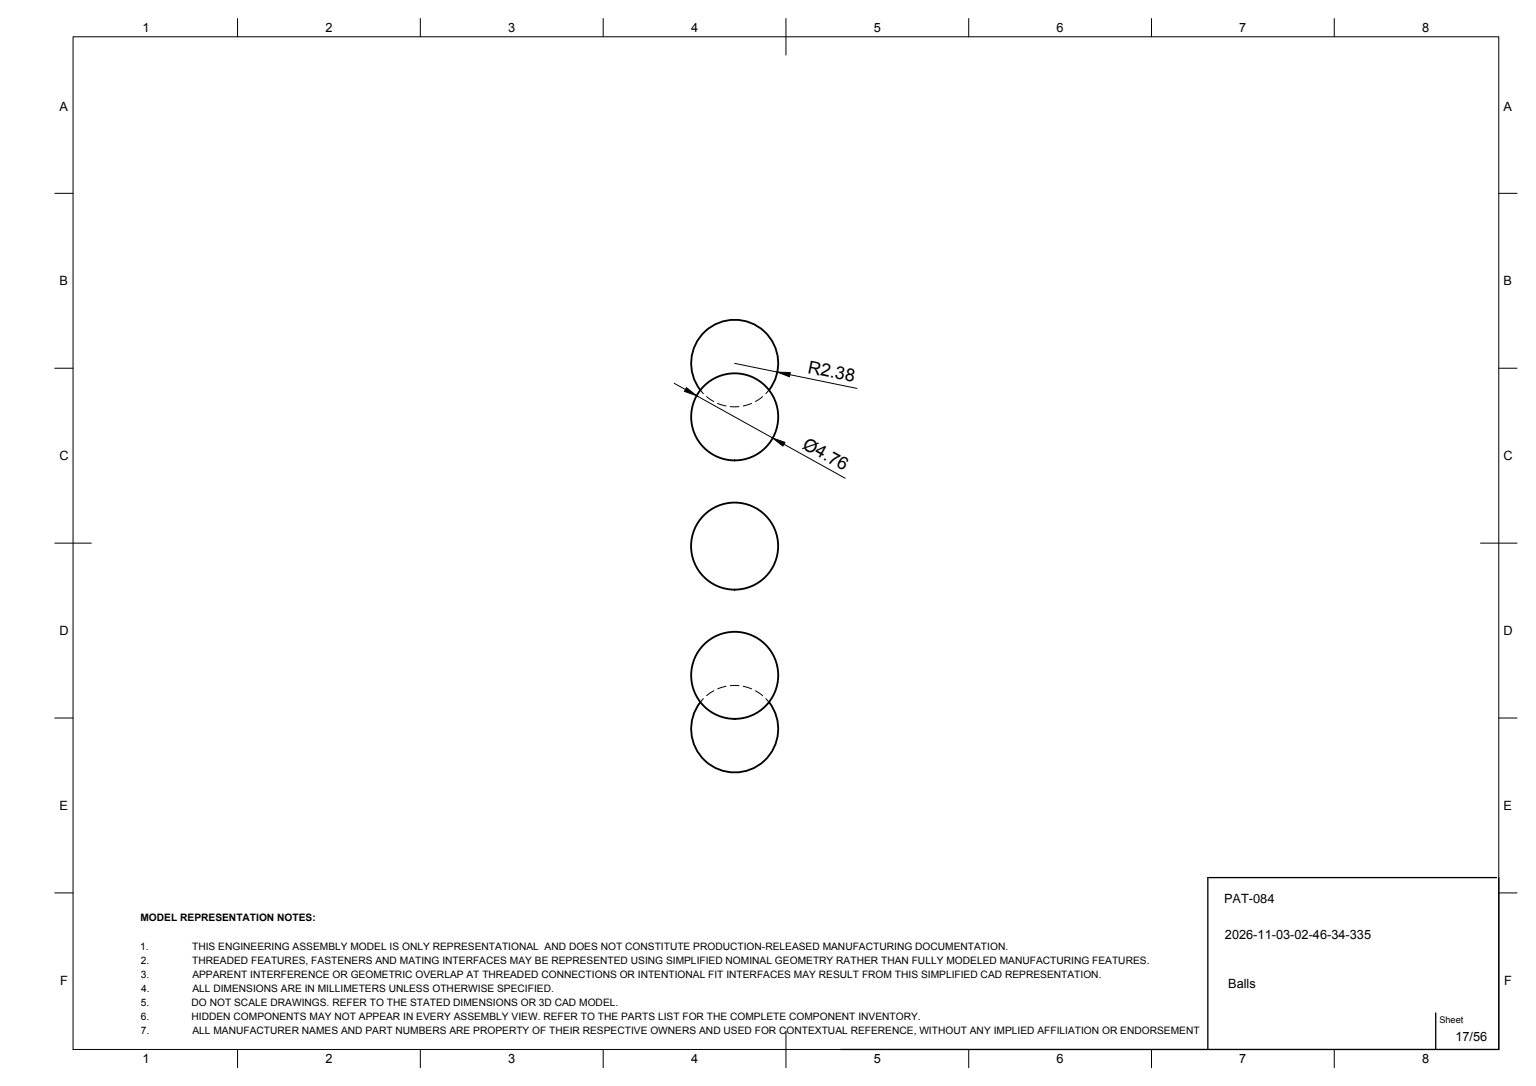
ISO-10303-21;
HEADER;
/* Generated by software containing ST-Developer
 * from STEP Tools, Inc. (www.steptools.com) 
 */

FILE_DESCRIPTION(
/* description */ ('Quick-return (Whitworth) mechanism'),
/* implementation_level */ '2;1');

FILE_NAME(
/* name */ 'Balls.step',
/* time_stamp */ '2026-10-28T03:25:57-07:00',
/* author */ (''),
/* organization */ (''),
/* preprocessor_version */ 'ST-DEVELOPER v20.2',
/* originating_system */ 'Autodesk Translation Framework v15.17.0.0',
/* authorisation */ '');

FILE_SCHEMA (('AUTOMOTIVE_DESIGN { 1 0 10303 214 3 1 1 }'));
ENDSEC;

DATA;
#10=MECHANICAL_DESIGN_GEOMETRIC_PRESENTATION_REPRESENTATION('',(#500,#501,#502,#503,#504,#505,#506,#507),#14878);
#333=SPHERICAL_SURFACE('',#8750,0.23815);
#334=SPHERICAL_SURFACE('',#8752,0.23815);
#335=SPHERICAL_SURFACE('',#8754,0.23815);
#336=SPHERICAL_SURFACE('',#8756,0.23815);
#337=SPHERICAL_SURFACE('',#8758,0.23815);
#338=SPHERICAL_SURFACE('',#8760,0.23815);
#339=SPHERICAL_SURFACE('',#8762,0.23815);
#340=SPHERICAL_SURFACE('',#8764,0.23815);
#412=SHAPE_REPRESENTATION_RELATIONSHIP('SRR','None',#15081,#456);
#456=ADVANCED_BREP_SHAPE_REPRESENTATION('',(#552,#553,#554,#555,#556,#557,
#558,#559),#14838);
#500=STYLED_ITEM('',(#15406),#552);
#501=STYLED_ITEM('',(#15406),#553);
#502=STYLED_ITEM('',(#15406),#554);
#503=STYLED_ITEM('',(#15406),#555);
#504=STYLED_ITEM('',(#15406),#556);
#505=STYLED_ITEM('',(#15406),#557);
#506=STYLED_ITEM('',(#15406),#558);
#507=STYLED_ITEM('',(#15406),#559);
#552=MANIFOLD_SOLID_BREP('Body1',#7854);
#553=MANIFOLD_SOLID_BREP('Body2',#7855);
#554=MANIFOLD_SOLID_BREP('Body3',#7856);
#555=MANIFOLD_SOLID_BREP('Body4',#7857);
#556=MANIFOLD_SOLID_BREP('Body5',#7858);
#557=MANIFOLD_SOLID_BREP('Body6',#7859);
#558=MANIFOLD_SOLID_BREP('Body7',#7860);
#559=MANIFOLD_SOLID_BREP('Body8',#7861);
#1213=FACE_OUTER_BOUND('',#1785,.T.);
#1214=FACE_OUTER_BOUND('',#1786,.T.);
#1215=FACE_OUTER_BOUND('',#1787,.T.);
#1216=FACE_OUTER_BOUND('',#1788,.T.);
#1217=FACE_OUTER_BOUND('',#1789,.T.);
#1218=FACE_OUTER_BOUND('',#1790,.T.);
#1219=FACE_OUTER_BOUND('',#1791,.T.);
#1220=FACE_OUTER_BOUND('',#1792,.T.);
#1785=EDGE_LOOP('',(#5982,#5983));
#1786=EDGE_LOOP('',(#5984,#5985));
#1787=EDGE_LOOP('',(#5986,#5987));
#1788=EDGE_LOOP('',(#5988,#5989));
#1789=EDGE_LOOP('',(#5990,#5991));
#1790=EDGE_LOOP('',(#5992,#5993));
#1791=EDGE_LOOP('',(#5994,#5995));
#1792=EDGE_LOOP('',(#5996,#5997));
#3402=CIRCLE('',#8751,0.23815);
#3403=CIRCLE('',#8753,0.23815);
#3404=CIRCLE('',#8755,0.23815);
#3405=CIRCLE('',#8757,0.23815);
#3406=CIRCLE('',#8759,0.23815);
#3407=CIRCLE('',#8761,0.23815);
#3408=CIRCLE('',#8763,0.23815);
#3409=CIRCLE('',#8765,0.23815);
#3871=VERTEX_POINT('',#12863);
#3872=VERTEX_POINT('',#12864);
#3873=VERTEX_POINT('',#12867);
#3874=VERTEX_POINT('',#12868);
#3875=VERTEX_POINT('',#12871);
#3876=VERTEX_POINT('',#12872);
#3877=VERTEX_POINT('',#12875);
#3878=VERTEX_POINT('',#12876);
#3879=VERTEX_POINT('',#12879);
#3880=VERTEX_POINT('',#12880);
#3881=VERTEX_POINT('',#12883);
#3882=VERTEX_POINT('',#12884);
#3883=VERTEX_POINT('',#12887);
#3884=VERTEX_POINT('',#12888);
#3885=VERTEX_POINT('',#12891);
#3886=VERTEX_POINT('',#12892);
#4648=EDGE_CURVE('',#3871,#3872,#3402,.T.);
#4649=EDGE_CURVE('',#3873,#3874,#3403,.T.);
#4650=EDGE_CURVE('',#3875,#3876,#3404,.T.);
#4651=EDGE_CURVE('',#3877,#3878,#3405,.T.);
#4652=EDGE_CURVE('',#3879,#3880,#3406,.T.);
#4653=EDGE_CURVE('',#3881,#3882,#3407,.T.);
#4654=EDGE_CURVE('',#3883,#3884,#3408,.T.);
#4655=EDGE_CURVE('',#3885,#3886,#3409,.T.);
#5982=ORIENTED_EDGE('',*,*,#4648,.T.);
#5983=ORIENTED_EDGE('',*,*,#4648,.F.);
#5984=ORIENTED_EDGE('',*,*,#4649,.T.);
#5985=ORIENTED_EDGE('',*,*,#4649,.F.);
#5986=ORIENTED_EDGE('',*,*,#4650,.T.);
#5987=ORIENTED_EDGE('',*,*,#4650,.F.);
#5988=ORIENTED_EDGE('',*,*,#4651,.T.);
#5989=ORIENTED_EDGE('',*,*,#4651,.F.);
#5990=ORIENTED_EDGE('',*,*,#4652,.T.);
#5991=ORIENTED_EDGE('',*,*,#4652,.F.);
#5992=ORIENTED_EDGE('',*,*,#4653,.T.);
#5993=ORIENTED_EDGE('',*,*,#4653,.F.);
#5994=ORIENTED_EDGE('',*,*,#4654,.T.);
#5995=ORIENTED_EDGE('',*,*,#4654,.F.);
#5996=ORIENTED_EDGE('',*,*,#4655,.T.);
#5997=ORIENTED_EDGE('',*,*,#4655,.F.);
#7544=ADVANCED_FACE('',(#1213),#333,.T.);
#7545=ADVANCED_FACE('',(#1214),#334,.T.);
#7546=ADVANCED_FACE('',(#1215),#335,.T.);
#7547=ADVANCED_FACE('',(#1216),#336,.T.);
#7548=ADVANCED_FACE('',(#1217),#337,.T.);
#7549=ADVANCED_FACE('',(#1218),#338,.T.);
#7550=ADVANCED_FACE('',(#1219),#339,.T.);
#7551=ADVANCED_FACE('',(#1220),#340,.T.);
#7854=CLOSED_SHELL('',(#7544));
#7855=CLOSED_SHELL('',(#7545));
#7856=CLOSED_SHELL('',(#7546));
#7857=CLOSED_SHELL('',(#7547));
#7858=CLOSED_SHELL('',(#7548));
#7859=CLOSED_SHELL('',(#7549));
#7860=CLOSED_SHELL('',(#7550));
#7861=CLOSED_SHELL('',(#7551));
#8749=AXIS2_PLACEMENT_3D('',#12861,#10293,#10294);
#8750=AXIS2_PLACEMENT_3D('',#12862,#10295,#10296);
#8751=AXIS2_PLACEMENT_3D('',#12865,#10297,#10298);
#8752=AXIS2_PLACEMENT_3D('',#12866,#10299,#10300);
#8753=AXIS2_PLACEMENT_3D('',#12869,#10301,#10302);
#8754=AXIS2_PLACEMENT_3D('',#12870,#10303,#10304);
#8755=AXIS2_PLACEMENT_3D('',#12873,#10305,#10306);
#8756=AXIS2_PLACEMENT_3D('',#12874,#10307,#10308);
#8757=AXIS2_PLACEMENT_3D('',#12877,#10309,#10310);
#8758=AXIS2_PLACEMENT_3D('',#12878,#10311,#10312);
#8759=AXIS2_PLACEMENT_3D('',#12881,#10313,#10314);
#8760=AXIS2_PLACEMENT_3D('',#12882,#10315,#10316);
#8761=AXIS2_PLACEMENT_3D('',#12885,#10317,#10318);
#8762=AXIS2_PLACEMENT_3D('',#12886,#10319,#10320);
#8763=AXIS2_PLACEMENT_3D('',#12889,#10321,#10322);
#8764=AXIS2_PLACEMENT_3D('',#12890,#10323,#10324);
#8765=AXIS2_PLACEMENT_3D('',#12893,#10325,#10326);
#10293=DIRECTION('axis',(0.,0.,1.));
#10294=DIRECTION('refdir',(1.,0.,0.));
#10295=DIRECTION('center_axis',(0.,0.,1.));
#10296=DIRECTION('ref_axis',(1.,0.,0.));
#10297=DIRECTION('center_axis',(1.22464679914735E-16,-1.,0.));
#10298=DIRECTION('ref_axis',(-1.,-1.22464679914735E-16,0.));
#10299=DIRECTION('center_axis',(0.707106781186548,0.,0.707106781186548));
#10300=DIRECTION('ref_axis',(0.707106781186548,0.,-0.707106781186548));
#10301=DIRECTION('center_axis',(8.65956056235494E-17,-1.,-8.65956056235493E-17));
#10302=DIRECTION('ref_axis',(-0.707106781186547,-1.22464679914735E-16,0.707106781186547));
#10303=DIRECTION('center_axis',(1.,0.,0.));
#10304=DIRECTION('ref_axis',(6.12323399573676E-17,0.,-1.));
#10305=DIRECTION('center_axis',(7.49879891330929E-33,-1.,-1.22464679914735E-16));
#10306=DIRECTION('ref_axis',(-6.12323399573676E-17,-1.22464679914735E-16,
1.));
#10307=DIRECTION('center_axis',(0.707106781186548,0.,-0.707106781186548));
#10308=DIRECTION('ref_axis',(-0.707106781186548,0.,-0.707106781186548));
#10309=DIRECTION('center_axis',(-8.65956056235493E-17,-1.,-8.65956056235494E-17));
#10310=DIRECTION('ref_axis',(0.707106781186547,-1.22464679914735E-16,0.707106781186547));
#10311=DIRECTION('center_axis',(0.,0.,-1.));
#10312=DIRECTION('ref_axis',(-1.,0.,-1.22464679914735E-16));
#10313=DIRECTION('center_axis',(-1.22464679914735E-16,-1.,-1.49975978266186E-32));
#10314=DIRECTION('ref_axis',(1.,-1.22464679914735E-16,1.22464679914735E-16));
#10315=DIRECTION('center_axis',(-0.707106781186547,0.,-0.707106781186548));
#10316=DIRECTION('ref_axis',(-0.707106781186548,0.,0.707106781186547));
#10317=DIRECTION('center_axis',(-8.65956056235493E-17,-1.,8.65956056235493E-17));
#10318=DIRECTION('ref_axis',(0.707106781186548,-1.22464679914735E-16,-0.707106781186547));
#10319=DIRECTION('center_axis',(-1.,0.,0.));
#10320=DIRECTION('ref_axis',(-1.83697019872103E-16,0.,1.));
#10321=DIRECTION('center_axis',(-2.24963967399279E-32,-1.,1.22464679914735E-16));
#10322=DIRECTION('ref_axis',(1.83697019872103E-16,-1.22464679914735E-16,
-1.));
#10323=DIRECTION('center_axis',(-0.707106781186548,0.,0.707106781186548));
#10324=DIRECTION('ref_axis',(0.707106781186547,0.,0.707106781186548));
#10325=DIRECTION('center_axis',(8.65956056235493E-17,-1.,8.65956056235493E-17));
#10326=DIRECTION('ref_axis',(-0.707106781186547,-1.22464679914735E-16,-0.707106781186548));
#12861=CARTESIAN_POINT('',(0.,0.,0.));
#12862=CARTESIAN_POINT('Origin',(1.,0.,0.));
#12863=CARTESIAN_POINT('',(1.,-1.78583896120461E-33,0.23815));
#12864=CARTESIAN_POINT('',(1.,-1.78583896120461E-33,-0.23815));
#12865=CARTESIAN_POINT('Origin',(1.,0.,0.));
#12866=CARTESIAN_POINT('Origin',(0.707106781186548,0.,-0.707106781186547));
#12867=CARTESIAN_POINT('',(0.875504261126124,-1.78583896120461E-33,-0.538709301246971));
#12868=CARTESIAN_POINT('',(0.538709301246971,-1.78583896120461E-33,-0.875504261126124));
#12869=CARTESIAN_POINT('Origin',(0.707106781186548,0.,-0.707106781186547));
#12870=CARTESIAN_POINT('Origin',(6.12323399573677E-17,0.,-1.));
#12871=CARTESIAN_POINT('',(0.23815,-1.78583896120461E-33,-1.));
#12872=CARTESIAN_POINT('',(-0.23815,-1.78583896120461E-33,-1.));
#12873=CARTESIAN_POINT('Origin',(6.12323399573677E-17,0.,-1.));
#12874=CARTESIAN_POINT('Origin',(-0.707106781186547,0.,-0.707106781186548));
#12875=CARTESIAN_POINT('',(-0.538709301246971,-1.78583896120461E-33,-0.875504261126124));
#12876=CARTESIAN_POINT('',(-0.875504261126124,-1.78583896120461E-33,-0.538709301246971));
#12877=CARTESIAN_POINT('Origin',(-0.707106781186547,0.,-0.707106781186548));
#12878=CARTESIAN_POINT('Origin',(-1.,0.,-1.22464679914735E-16));
#12879=CARTESIAN_POINT('',(-1.,-1.78583896120461E-33,-0.23815));
#12880=CARTESIAN_POINT('',(-1.,-1.78583896120461E-33,0.23815));
#12881=CARTESIAN_POINT('Origin',(-1.,0.,-1.22464679914735E-16));
#12882=CARTESIAN_POINT('Origin',(-0.707106781186548,0.,0.707106781186547));
#12883=CARTESIAN_POINT('',(-0.875504261126124,-7.94881478324376E-33,0.538709301246971));
#12884=CARTESIAN_POINT('',(-0.538709301246971,4.37713686083455E-33,0.875504261126124));
#12885=CARTESIAN_POINT('Origin',(-0.707106781186548,0.,0.707106781186547));
#12886=CARTESIAN_POINT('Origin',(-1.83697019872103E-16,0.,1.));
#12887=CARTESIAN_POINT('',(-0.23815,-1.78583896120461E-33,1.));
#12888=CARTESIAN_POINT('',(0.23815,-1.78583896120461E-33,1.));
#12889=CARTESIAN_POINT('Origin',(-1.83697019872103E-16,0.,1.));
#12890=CARTESIAN_POINT('Origin',(0.707106781186547,0.,0.707106781186548));
#12891=CARTESIAN_POINT('',(0.538709301246971,-4.86732687222419E-33,0.875504261126124));
#12892=CARTESIAN_POINT('',(0.875504261126124,1.29564894981497E-33,0.538709301246971));
#12893=CARTESIAN_POINT('Origin',(0.707106781186547,0.,0.707106781186548));
#14784=UNCERTAINTY_MEASURE_WITH_UNIT(LENGTH_MEASURE(0.001),#14879,
'DISTANCE_ACCURACY_VALUE',
'Maximum model space distance between geometric entities at asserted c
onnectivities');
#14824=UNCERTAINTY_MEASURE_WITH_UNIT(LENGTH_MEASURE(0.001),#14879,
'DISTANCE_ACCURACY_VALUE',
'Maximum model space distance between geometric entities at asserted c
onnectivities');
#14838=(
GEOMETRIC_REPRESENTATION_CONTEXT(3)
GLOBAL_UNCERTAINTY_ASSIGNED_CONTEXT((#14784))
GLOBAL_UNIT_ASSIGNED_CONTEXT((#14879,#14881,#14882))
REPRESENTATION_CONTEXT('','3D')
);
#14878=(
GEOMETRIC_REPRESENTATION_CONTEXT(3)
GLOBAL_UNCERTAINTY_ASSIGNED_CONTEXT((#14824))
GLOBAL_UNIT_ASSIGNED_CONTEXT((#14879,#14881,#14882))
REPRESENTATION_CONTEXT('','3D')
);
#14879=(
LENGTH_UNIT()
NAMED_UNIT(*)
SI_UNIT(.CENTI.,.METRE.)
);
#14881=(
NAMED_UNIT(*)
PLANE_ANGLE_UNIT()
SI_UNIT($,.RADIAN.)
);
#14882=(
NAMED_UNIT(*)
SI_UNIT($,.STERADIAN.)
SOLID_ANGLE_UNIT()
);
#14896=SHAPE_DEFINITION_REPRESENTATION(#14949,#15081);
#14949=PRODUCT_DEFINITION_SHAPE('',$,#15135);
#15081=SHAPE_REPRESENTATION('',(#8749),#14838);
#15121=PRODUCT_DEFINITION_CONTEXT('part definition',#15282,'design');
#15135=PRODUCT_DEFINITION('Balls','Balls',#15188,#15121);
#15188=PRODUCT_DEFINITION_FORMATION('',$,#15297);
#15282=APPLICATION_CONTEXT(
'Core Data for Automotive Mechanical Design Process');
#15283=PRODUCT_CONTEXT('part definition',#15282,'mechanical');
#15297=PRODUCT('Balls','Balls','Balls',(#15283));
#15400=COLOUR_RGB('Grey',0.48,0.52,0.57);
#15401=FILL_AREA_STYLE_COLOUR('',#15400);
#15402=FILL_AREA_STYLE('',(#15401));
#15403=SURFACE_STYLE_FILL_AREA(#15402);
#15404=SURFACE_SIDE_STYLE('',(#15403));
#15405=SURFACE_STYLE_USAGE(.BOTH.,#15404);
#15406=PRESENTATION_STYLE_ASSIGNMENT((#15405));
ENDSEC;
END-ISO-10303-21;
